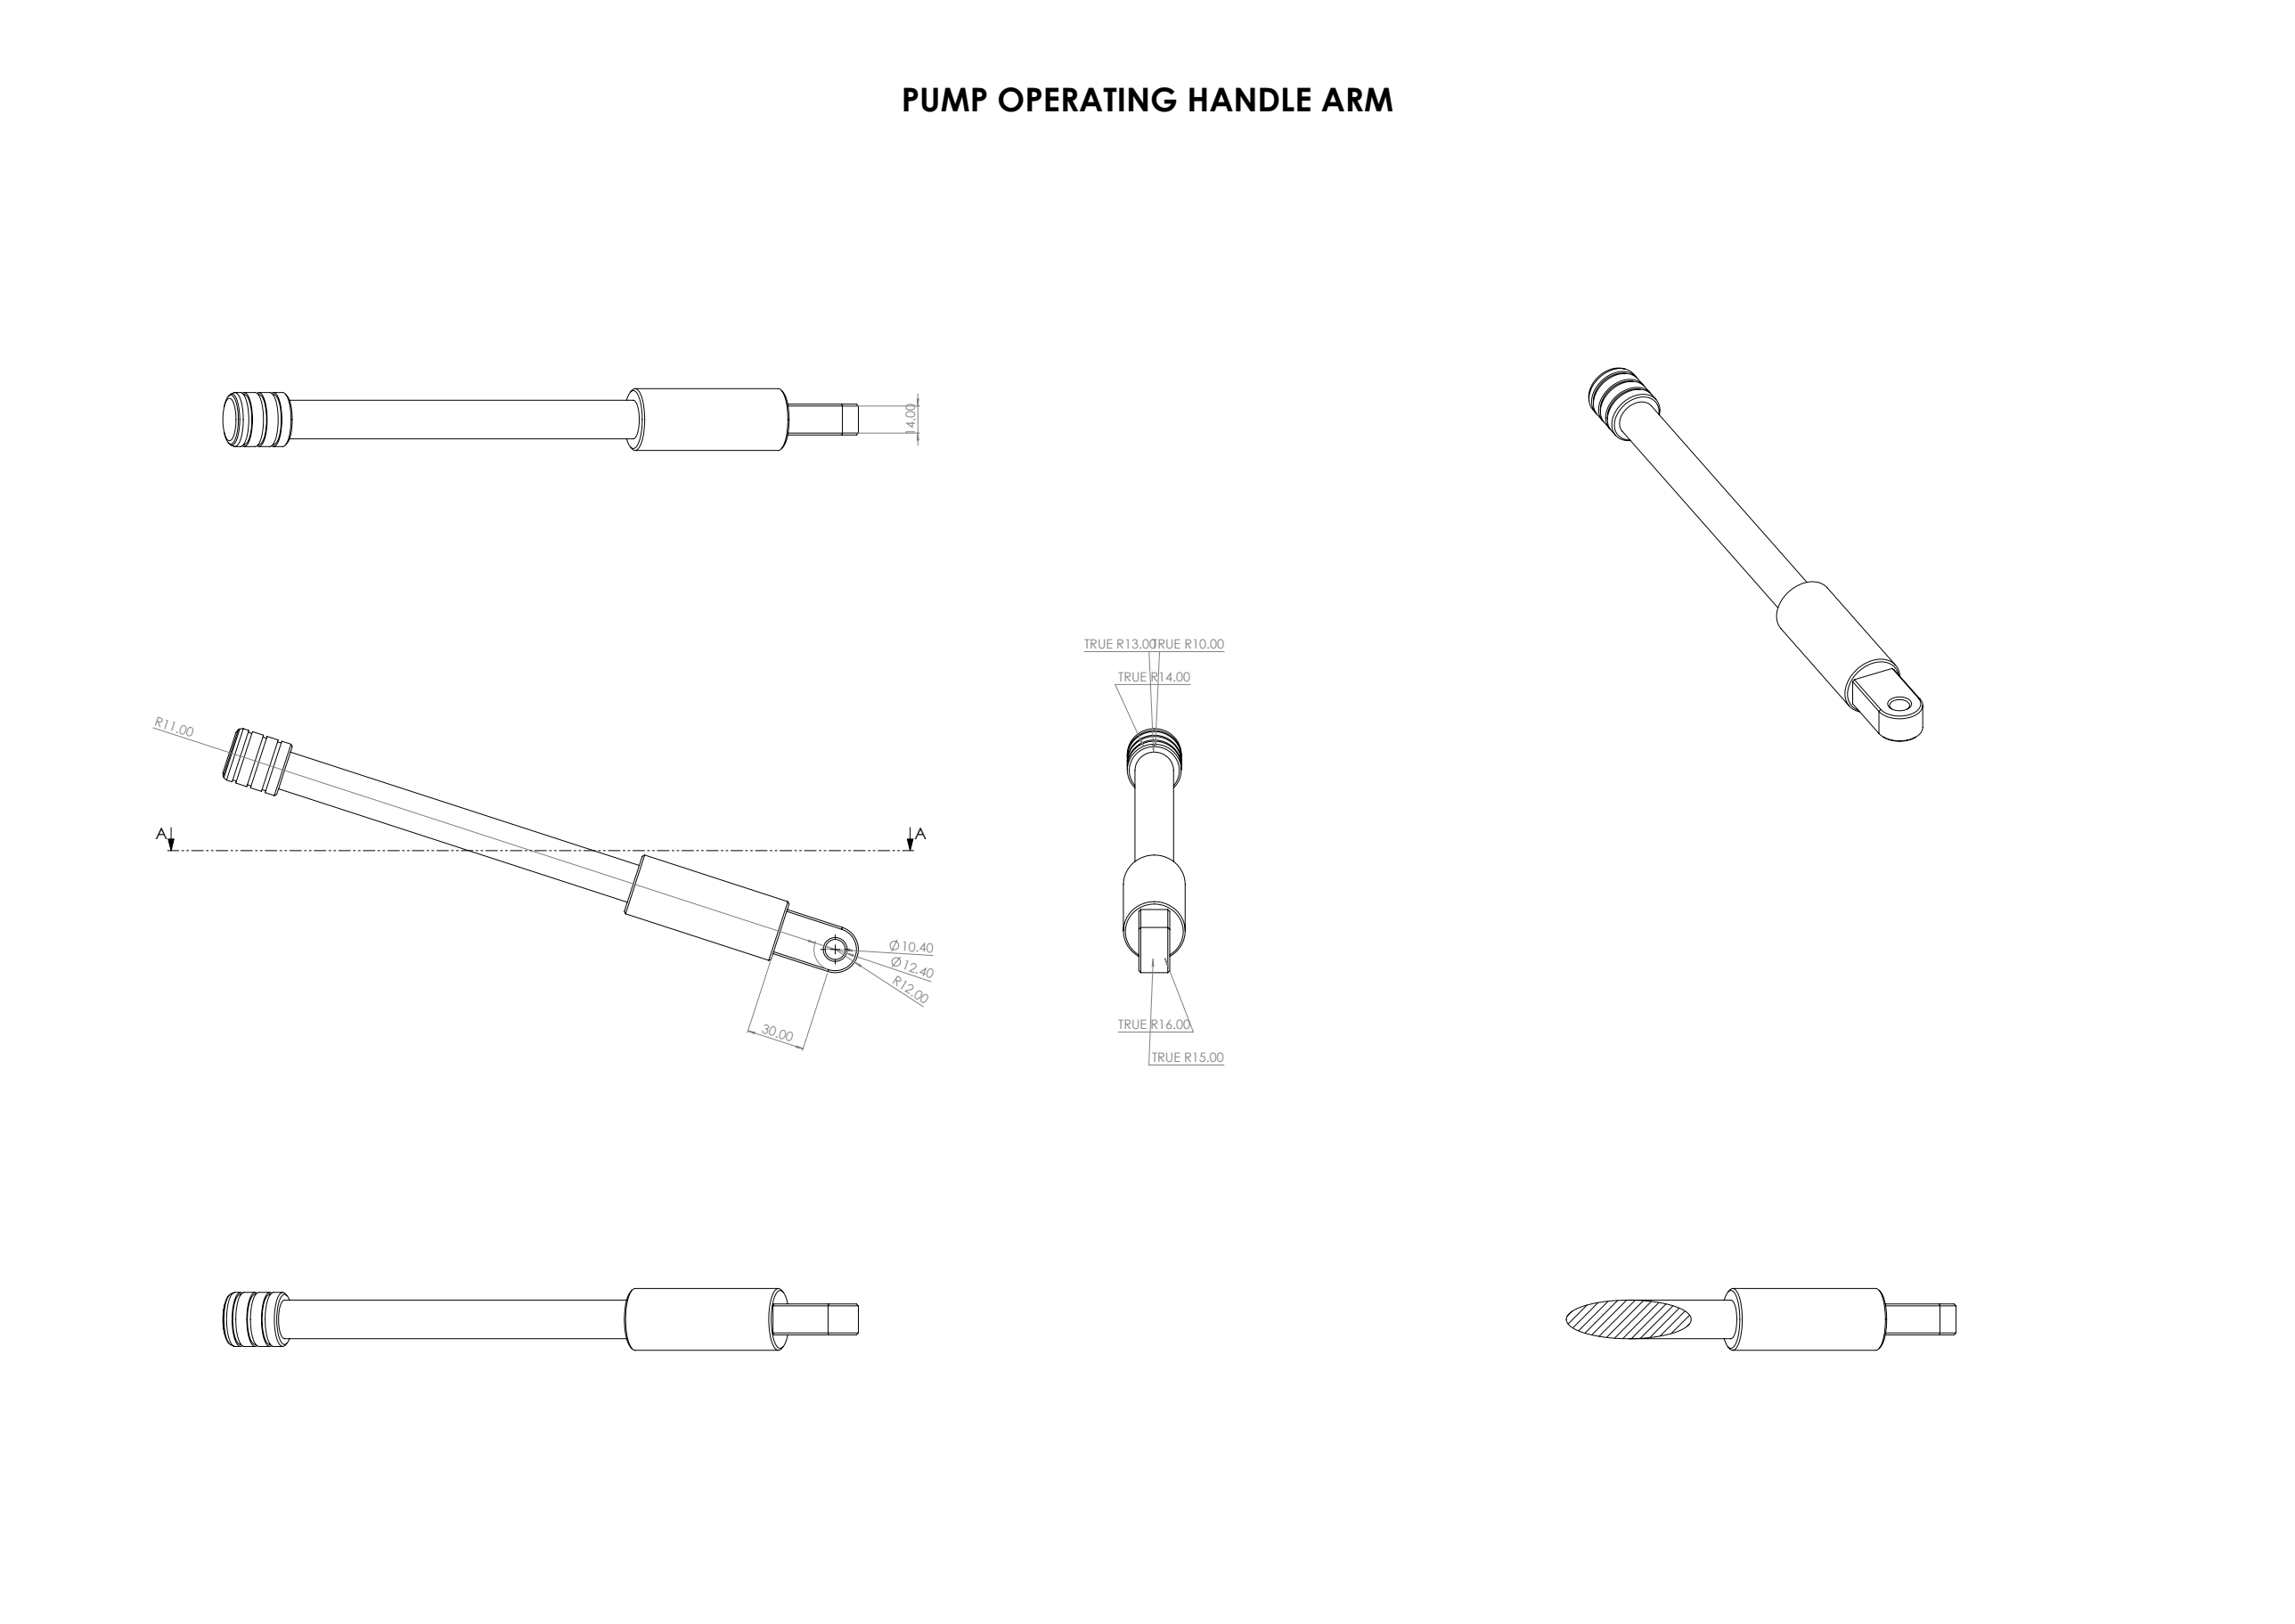
ISO-10303-21;
HEADER;
/* Generated by software containing ST-Developer
 * from STEP Tools, Inc. (www.steptools.com) 
 */

FILE_DESCRIPTION(
/* description */ (''),
/* implementation_level */ '2;1');

FILE_NAME(
/* name */ '11_Pump_Operating_Handle_Arm.step',
/* time_stamp */ '2026-10-20T10:03:03-07:00',
/* author */ (''),
/* organization */ (''),
/* preprocessor_version */ 'ST-DEVELOPER v20.2',
/* originating_system */ 'Autodesk Translation Framework v15.15.0.0',
/* authorisation */ '');

FILE_SCHEMA (('AUTOMOTIVE_DESIGN { 1 0 10303 214 3 1 1 }'));
ENDSEC;

DATA;
#10=MECHANICAL_DESIGN_GEOMETRIC_PRESENTATION_REPRESENTATION('',(#542,#543,#544,#545,#546,#547,#548,#549),#71492);
#399=SHAPE_REPRESENTATION_RELATIONSHIP('SRR','None',#71620,#418);
#418=ADVANCED_BREP_SHAPE_REPRESENTATION('',(#437),#71490);
#437=MANIFOLD_SOLID_BREP('Handle',#28476);
#542=STYLED_ITEM('',(#71880),#28308);
#543=STYLED_ITEM('',(#71880),#28315);
#544=STYLED_ITEM('',(#71880),#28318);
#545=STYLED_ITEM('',(#71880),#28320);
#546=STYLED_ITEM('',(#71880),#28322);
#547=STYLED_ITEM('',(#71880),#28324);
#548=STYLED_ITEM('',(#71880),#28326);
#549=STYLED_ITEM('',(#71880),#437);
#1833=CYLINDRICAL_SURFACE('',#30489,1.40000000000001);
#1834=CYLINDRICAL_SURFACE('',#30494,0.52);
#1835=CYLINDRICAL_SURFACE('',#30506,1.40000000000001);
#1836=CYLINDRICAL_SURFACE('',#30512,1.30000000000003);
#1837=CYLINDRICAL_SURFACE('',#30516,1.40000000000001);
#1838=CYLINDRICAL_SURFACE('',#30520,1.3);
#1839=CYLINDRICAL_SURFACE('',#30524,1.40000000000001);
#1840=CYLINDRICAL_SURFACE('',#30528,1.30000000000003);
#1841=CYLINDRICAL_SURFACE('',#30535,1.60000000000001);
#1842=CYLINDRICAL_SURFACE('',#30541,0.999999999999985);
#1843=CYLINDRICAL_SURFACE('',#30548,1.19999999999999);
#1988=FACE_BOUND('',#6098,.T.);
#1989=FACE_BOUND('',#6101,.T.);
#1990=FACE_BOUND('',#6105,.T.);
#1991=FACE_BOUND('',#6107,.T.);
#1992=FACE_BOUND('',#6110,.T.);
#1993=FACE_BOUND('',#6113,.T.);
#1994=FACE_BOUND('',#6116,.T.);
#1995=FACE_BOUND('',#6119,.T.);
#1996=FACE_BOUND('',#6122,.T.);
#1997=FACE_BOUND('',#6124,.T.);
#1998=FACE_BOUND('',#6129,.T.);
#2575=CIRCLE('',#30479,1.1);
#2576=CIRCLE('',#30480,1.27071067811866);
#2577=CIRCLE('',#30481,1.27071067811866);
#2578=CIRCLE('',#30483,1.32928932188137);
#2579=CIRCLE('',#30484,1.32928932188137);
#2580=CIRCLE('',#30487,1.40000000000001);
#2581=CIRCLE('',#30488,1.40000000000001);
#2582=CIRCLE('',#30490,1.40000000000001);
#2583=CIRCLE('',#30492,0.619999999999999);
#2584=CIRCLE('',#30493,0.52);
#2585=CIRCLE('',#30495,0.52);
#2586=CIRCLE('',#30497,1.09999999999999);
#2587=CIRCLE('',#30499,0.619999999999999);
#2588=CIRCLE('',#30501,1.09999999999999);
#2589=CIRCLE('',#30503,1.40000000000001);
#2590=CIRCLE('',#30504,1.40000000000001);
#2591=CIRCLE('',#30505,1.30000000000001);
#2592=CIRCLE('',#30507,1.40000000000001);
#2593=CIRCLE('',#30509,1.);
#2594=CIRCLE('',#30511,1.30000000000002);
#2595=CIRCLE('',#30513,1.30000000000002);
#2596=CIRCLE('',#30515,1.40000000000001);
#2597=CIRCLE('',#30517,1.40000000000001);
#2598=CIRCLE('',#30519,1.29999999999999);
#2599=CIRCLE('',#30521,1.29999999999999);
#2600=CIRCLE('',#30523,1.40000000000001);
#2601=CIRCLE('',#30525,1.40000000000001);
#2602=CIRCLE('',#30527,1.30000000000002);
#2603=CIRCLE('',#30529,1.30000000000002);
#2604=CIRCLE('',#30532,1.5);
#2605=CIRCLE('',#30534,1.6);
#2606=CIRCLE('',#30536,1.60000000000002);
#2607=CIRCLE('',#30538,1.5);
#2608=CIRCLE('',#30540,0.999999999999996);
#2609=CIRCLE('',#30546,1.19999999999999);
#2610=CIRCLE('',#30549,1.19999999999999);
#2901=CONICAL_SURFACE('',#30478,1.18535533905933,1.17809724509622);
#2902=CONICAL_SURFACE('',#30482,1.30000000000001,0.78539816339746);
#2903=CONICAL_SURFACE('',#30486,1.36464466094069,0.392699081698615);
#2904=CONICAL_SURFACE('',#30491,0.569999999999999,0.785398163397448);
#2905=CONICAL_SURFACE('',#30498,0.569999999999999,0.785398163397448);
#2906=CONICAL_SURFACE('',#30502,1.35000000000001,0.785398163397418);
#2907=CONICAL_SURFACE('',#30533,1.54999999999999,0.785398163397423);
#2908=CONICAL_SURFACE('',#30537,1.54999999999999,0.785398163397517);
#2909=CONICAL_SURFACE('',#30545,1.14999999999999,0.785398163397454);
#2910=CONICAL_SURFACE('',#30551,1.14999999999999,0.785398163397454);
#4396=FACE_OUTER_BOUND('',#6090,.T.);
#4397=FACE_OUTER_BOUND('',#6091,.T.);
#4398=FACE_OUTER_BOUND('',#6092,.T.);
#4399=FACE_OUTER_BOUND('',#6093,.T.);
#4400=FACE_OUTER_BOUND('',#6094,.T.);
#4401=FACE_OUTER_BOUND('',#6095,.T.);
#4402=FACE_OUTER_BOUND('',#6096,.T.);
#4403=FACE_OUTER_BOUND('',#6097,.T.);
#4404=FACE_OUTER_BOUND('',#6099,.T.);
#4405=FACE_OUTER_BOUND('',#6100,.T.);
#4406=FACE_OUTER_BOUND('',#6102,.T.);
#4407=FACE_OUTER_BOUND('',#6103,.T.);
#4408=FACE_OUTER_BOUND('',#6104,.T.);
#4409=FACE_OUTER_BOUND('',#6106,.T.);
#4410=FACE_OUTER_BOUND('',#6108,.T.);
#4411=FACE_OUTER_BOUND('',#6109,.T.);
#4412=FACE_OUTER_BOUND('',#6111,.T.);
#4413=FACE_OUTER_BOUND('',#6112,.T.);
#4414=FACE_OUTER_BOUND('',#6114,.T.);
#4415=FACE_OUTER_BOUND('',#6115,.T.);
#4416=FACE_OUTER_BOUND('',#6117,.T.);
#4417=FACE_OUTER_BOUND('',#6118,.T.);
#4418=FACE_OUTER_BOUND('',#6120,.T.);
#4419=FACE_OUTER_BOUND('',#6121,.T.);
#4420=FACE_OUTER_BOUND('',#6123,.T.);
#4421=FACE_OUTER_BOUND('',#6125,.T.);
#4422=FACE_OUTER_BOUND('',#6126,.T.);
#4423=FACE_OUTER_BOUND('',#6127,.T.);
#4424=FACE_OUTER_BOUND('',#6128,.T.);
#4425=FACE_OUTER_BOUND('',#6130,.T.);
#4426=FACE_OUTER_BOUND('',#6131,.T.);
#4427=FACE_OUTER_BOUND('',#6132,.T.);
#4428=FACE_OUTER_BOUND('',#6133,.T.);
#4429=FACE_OUTER_BOUND('',#6134,.T.);
#4430=FACE_OUTER_BOUND('',#6135,.T.);
#4431=FACE_OUTER_BOUND('',#6136,.T.);
#4432=FACE_OUTER_BOUND('',#6137,.T.);
#4433=FACE_OUTER_BOUND('',#6138,.T.);
#4434=FACE_OUTER_BOUND('',#6139,.T.);
#6090=EDGE_LOOP('',(#25387,#25388,#25389,#25390,#25391));
#6091=EDGE_LOOP('',(#25392,#25393,#25394,#25395,#25396,#25397));
#6092=EDGE_LOOP('',(#25398));
#6093=EDGE_LOOP('',(#25399,#25400,#25401,#25402,#25403,#25404));
#6094=EDGE_LOOP('',(#25405,#25406,#25407,#25408,#25409));
#6095=EDGE_LOOP('',(#25410,#25411,#25412,#25413));
#6096=EDGE_LOOP('',(#25414,#25415,#25416,#25417));
#6097=EDGE_LOOP('',(#25418,#25419,#25420,#25421));
#6098=EDGE_LOOP('',(#25422));
#6099=EDGE_LOOP('',(#25423,#25424,#25425,#25426));
#6100=EDGE_LOOP('',(#25427,#25428,#25429,#25430));
#6101=EDGE_LOOP('',(#25431));
#6102=EDGE_LOOP('',(#25432,#25433,#25434,#25435,#25436));
#6103=EDGE_LOOP('',(#25437,#25438,#25439,#25440,#25441));
#6104=EDGE_LOOP('',(#25442));
#6105=EDGE_LOOP('',(#25443));
#6106=EDGE_LOOP('',(#25444));
#6107=EDGE_LOOP('',(#25445));
#6108=EDGE_LOOP('',(#25446,#25447,#25448,#25449));
#6109=EDGE_LOOP('',(#25450));
#6110=EDGE_LOOP('',(#25451));
#6111=EDGE_LOOP('',(#25452,#25453,#25454,#25455));
#6112=EDGE_LOOP('',(#25456));
#6113=EDGE_LOOP('',(#25457));
#6114=EDGE_LOOP('',(#25458,#25459,#25460,#25461));
#6115=EDGE_LOOP('',(#25462));
#6116=EDGE_LOOP('',(#25463));
#6117=EDGE_LOOP('',(#25464,#25465,#25466,#25467));
#6118=EDGE_LOOP('',(#25468));
#6119=EDGE_LOOP('',(#25469));
#6120=EDGE_LOOP('',(#25470,#25471,#25472,#25473));
#6121=EDGE_LOOP('',(#25474));
#6122=EDGE_LOOP('',(#25475));
#6123=EDGE_LOOP('',(#25476));
#6124=EDGE_LOOP('',(#25477,#25478,#25479,#25480,#25481,#25482,#25483,#25484));
#6125=EDGE_LOOP('',(#25485,#25486,#25487,#25488));
#6126=EDGE_LOOP('',(#25489,#25490,#25491,#25492));
#6127=EDGE_LOOP('',(#25493,#25494,#25495,#25496));
#6128=EDGE_LOOP('',(#25497));
#6129=EDGE_LOOP('',(#25498));
#6130=EDGE_LOOP('',(#25499,#25500,#25501,#25502));
#6131=EDGE_LOOP('',(#25503,#25504,#25505,#25506));
#6132=EDGE_LOOP('',(#25507,#25508,#25509,#25510));
#6133=EDGE_LOOP('',(#25511,#25512,#25513,#25514));
#6134=EDGE_LOOP('',(#25515,#25516,#25517,#25518));
#6135=EDGE_LOOP('',(#25519,#25520,#25521,#25522));
#6136=EDGE_LOOP('',(#25523,#25524,#25525,#25526));
#6137=EDGE_LOOP('',(#25527,#25528,#25529,#25530));
#6138=EDGE_LOOP('',(#25531,#25532,#25533,#25534));
#6139=EDGE_LOOP('',(#25535,#25536,#25537,#25538));
#8604=LINE('',#70692,#11092);
#8605=LINE('',#70698,#11093);
#8606=LINE('',#70705,#11094);
#8607=LINE('',#70711,#11095);
#8608=LINE('',#70717,#11096);
#8609=LINE('',#70722,#11097);
#8610=LINE('',#70726,#11098);
#8611=LINE('',#70728,#11099);
#8612=LINE('',#70731,#11100);
#8613=LINE('',#70735,#11101);
#8614=LINE('',#70739,#11102);
#8615=LINE('',#70741,#11103);
#8616=LINE('',#70744,#11104);
#8617=LINE('',#70751,#11105);
#8618=LINE('',#70756,#11106);
#8619=LINE('',#70766,#11107);
#8620=LINE('',#70772,#11108);
#8621=LINE('',#70780,#11109);
#8622=LINE('',#70786,#11110);
#8623=LINE('',#70794,#11111);
#8624=LINE('',#70800,#11112);
#8625=LINE('',#70802,#11113);
#8626=LINE('',#70804,#11114);
#8627=LINE('',#70805,#11115);
#8628=LINE('',#70807,#11116);
#8629=LINE('',#70808,#11117);
#8630=LINE('',#70812,#11118);
#8631=LINE('',#70816,#11119);
#8632=LINE('',#70820,#11120);
#8633=LINE('',#70825,#11121);
#8634=LINE('',#70828,#11122);
#8635=LINE('',#70829,#11123);
#8636=LINE('',#70832,#11124);
#8637=LINE('',#70833,#11125);
#8638=LINE('',#70835,#11126);
#8639=LINE('',#70838,#11127);
#8640=LINE('',#70841,#11128);
#8641=LINE('',#70845,#11129);
#8642=LINE('',#70847,#11130);
#8643=LINE('',#70848,#11131);
#11092=VECTOR('',#36741,1.18535533905933);
#11093=VECTOR('',#36748,1.30000000000001);
#11094=VECTOR('',#36757,1.36464466094067);
#11095=VECTOR('',#36764,1.40000000000001);
#11096=VECTOR('',#36771,0.57);
#11097=VECTOR('',#36778,0.52);
#11098=VECTOR('',#36781,1.);
#11099=VECTOR('',#36782,1.);
#11100=VECTOR('',#36785,1.);
#11101=VECTOR('',#36790,0.57);
#11102=VECTOR('',#36793,1.);
#11103=VECTOR('',#36794,1.);
#11104=VECTOR('',#36797,1.);
#11105=VECTOR('',#36804,1.35000000000004);
#11106=VECTOR('',#36811,1.40000000000001);
#11107=VECTOR('',#36824,1.30000000000003);
#11108=VECTOR('',#36831,1.40000000000001);
#11109=VECTOR('',#36842,1.3);
#11110=VECTOR('',#36849,1.40000000000001);
#11111=VECTOR('',#36860,1.30000000000003);
#11112=VECTOR('',#36867,1.);
#11113=VECTOR('',#36868,1.);
#11114=VECTOR('',#36869,1.);
#11115=VECTOR('',#36870,1.);
#11116=VECTOR('',#36871,1.);
#11117=VECTOR('',#36872,1.);
#11118=VECTOR('',#36877,1.54999999999999);
#11119=VECTOR('',#36882,1.60000000000001);
#11120=VECTOR('',#36887,1.54999999999999);
#11121=VECTOR('',#36894,0.999999999999985);
#11122=VECTOR('',#36897,1.);
#11123=VECTOR('',#36898,1.);
#11124=VECTOR('',#36901,1.);
#11125=VECTOR('',#36902,1.);
#11126=VECTOR('',#36905,1.);
#11127=VECTOR('',#36908,1.);
#11128=VECTOR('',#36913,1.);
#11129=VECTOR('',#36918,1.);
#11130=VECTOR('',#36921,1.);
#11131=VECTOR('',#36922,1.);
#13643=VERTEX_POINT('',#70689);
#13644=VERTEX_POINT('',#70691);
#13645=VERTEX_POINT('',#70693);
#13646=VERTEX_POINT('',#70697);
#13647=VERTEX_POINT('',#70699);
#13648=VERTEX_POINT('',#70704);
#13649=VERTEX_POINT('',#70706);
#13650=VERTEX_POINT('',#70710);
#13651=VERTEX_POINT('',#70714);
#13652=VERTEX_POINT('',#70716);
#13653=VERTEX_POINT('',#70720);
#13654=VERTEX_POINT('',#70724);
#13655=VERTEX_POINT('',#70725);
#13656=VERTEX_POINT('',#70727);
#13657=VERTEX_POINT('',#70729);
#13658=VERTEX_POINT('',#70733);
#13659=VERTEX_POINT('',#70737);
#13660=VERTEX_POINT('',#70738);
#13661=VERTEX_POINT('',#70740);
#13662=VERTEX_POINT('',#70742);
#13663=VERTEX_POINT('',#70746);
#13664=VERTEX_POINT('',#70747);
#13665=VERTEX_POINT('',#70750);
#13666=VERTEX_POINT('',#70754);
#13667=VERTEX_POINT('',#70758);
#13668=VERTEX_POINT('',#70761);
#13669=VERTEX_POINT('',#70764);
#13670=VERTEX_POINT('',#70768);
#13671=VERTEX_POINT('',#70771);
#13672=VERTEX_POINT('',#70775);
#13673=VERTEX_POINT('',#70778);
#13674=VERTEX_POINT('',#70782);
#13675=VERTEX_POINT('',#70785);
#13676=VERTEX_POINT('',#70789);
#13677=VERTEX_POINT('',#70792);
#13678=VERTEX_POINT('',#70797);
#13679=VERTEX_POINT('',#70799);
#13680=VERTEX_POINT('',#70801);
#13681=VERTEX_POINT('',#70803);
#13682=VERTEX_POINT('',#70806);
#13683=VERTEX_POINT('',#70810);
#13684=VERTEX_POINT('',#70814);
#13685=VERTEX_POINT('',#70818);
#13686=VERTEX_POINT('',#70822);
#13687=VERTEX_POINT('',#70827);
#13688=VERTEX_POINT('',#70831);
#13689=VERTEX_POINT('',#70837);
#13690=VERTEX_POINT('',#70843);
#17577=EDGE_CURVE('',#13643,#13643,#2575,.T.);
#17578=EDGE_CURVE('',#13643,#13644,#8604,.T.);
#17579=EDGE_CURVE('',#13644,#13645,#2576,.T.);
#17580=EDGE_CURVE('',#13645,#13644,#2577,.T.);
#17581=EDGE_CURVE('',#13645,#13646,#8605,.T.);
#17582=EDGE_CURVE('',#13647,#13646,#2578,.T.);
#17583=EDGE_CURVE('',#13646,#13647,#2579,.T.);
#17584=EDGE_CURVE('',#13647,#13648,#8606,.T.);
#17585=EDGE_CURVE('',#13648,#13649,#2580,.T.);
#17586=EDGE_CURVE('',#13649,#13648,#2581,.T.);
#17587=EDGE_CURVE('',#13649,#13650,#8607,.T.);
#17588=EDGE_CURVE('',#13650,#13650,#2582,.T.);
#17589=EDGE_CURVE('',#13651,#13651,#2583,.T.);
#17590=EDGE_CURVE('',#13651,#13652,#8608,.T.);
#17591=EDGE_CURVE('',#13652,#13652,#2584,.T.);
#17592=EDGE_CURVE('',#13653,#13653,#2585,.T.);
#17593=EDGE_CURVE('',#13653,#13652,#8609,.T.);
#17594=EDGE_CURVE('',#13654,#13655,#8610,.T.);
#17595=EDGE_CURVE('',#13656,#13655,#8611,.T.);
#17596=EDGE_CURVE('',#13657,#13656,#2586,.T.);
#17597=EDGE_CURVE('',#13654,#13657,#8612,.T.);
#17598=EDGE_CURVE('',#13658,#13658,#2587,.T.);
#17599=EDGE_CURVE('',#13658,#13653,#8613,.T.);
#17600=EDGE_CURVE('',#13659,#13660,#8614,.T.);
#17601=EDGE_CURVE('',#13661,#13660,#8615,.T.);
#17602=EDGE_CURVE('',#13662,#13661,#2588,.T.);
#17603=EDGE_CURVE('',#13659,#13662,#8616,.T.);
#17604=EDGE_CURVE('',#13663,#13664,#2589,.T.);
#17605=EDGE_CURVE('',#13664,#13663,#2590,.T.);
#17606=EDGE_CURVE('',#13663,#13665,#8617,.T.);
#17607=EDGE_CURVE('',#13665,#13665,#2591,.T.);
#17608=EDGE_CURVE('',#13666,#13666,#2592,.T.);
#17609=EDGE_CURVE('',#13666,#13664,#8618,.T.);
#17610=EDGE_CURVE('',#13667,#13667,#2593,.T.);
#17611=EDGE_CURVE('',#13668,#13668,#2594,.T.);
#17612=EDGE_CURVE('',#13669,#13669,#2595,.T.);
#17613=EDGE_CURVE('',#13669,#13668,#8619,.T.);
#17614=EDGE_CURVE('',#13670,#13670,#2596,.T.);
#17615=EDGE_CURVE('',#13670,#13671,#8620,.T.);
#17616=EDGE_CURVE('',#13671,#13671,#2597,.T.);
#17617=EDGE_CURVE('',#13672,#13672,#2598,.T.);
#17618=EDGE_CURVE('',#13673,#13673,#2599,.T.);
#17619=EDGE_CURVE('',#13673,#13672,#8621,.T.);
#17620=EDGE_CURVE('',#13674,#13674,#2600,.T.);
#17621=EDGE_CURVE('',#13674,#13675,#8622,.T.);
#17622=EDGE_CURVE('',#13675,#13675,#2601,.T.);
#17623=EDGE_CURVE('',#13676,#13676,#2602,.T.);
#17624=EDGE_CURVE('',#13677,#13677,#2603,.T.);
#17625=EDGE_CURVE('',#13677,#13676,#8623,.T.);
#17626=EDGE_CURVE('',#13678,#13678,#2604,.T.);
#17627=EDGE_CURVE('',#13660,#13679,#8624,.T.);
#17628=EDGE_CURVE('',#13680,#13659,#8625,.T.);
#17629=EDGE_CURVE('',#13681,#13680,#8626,.T.);
#17630=EDGE_CURVE('',#13655,#13681,#8627,.T.);
#17631=EDGE_CURVE('',#13682,#13654,#8628,.T.);
#17632=EDGE_CURVE('',#13679,#13682,#8629,.T.);
#17633=EDGE_CURVE('',#13683,#13683,#2605,.T.);
#17634=EDGE_CURVE('',#13683,#13678,#8630,.T.);
#17635=EDGE_CURVE('',#13684,#13684,#2606,.T.);
#17636=EDGE_CURVE('',#13684,#13683,#8631,.T.);
#17637=EDGE_CURVE('',#13685,#13685,#2607,.T.);
#17638=EDGE_CURVE('',#13685,#13684,#8632,.T.);
#17639=EDGE_CURVE('',#13686,#13686,#2608,.T.);
#17640=EDGE_CURVE('',#13667,#13686,#8633,.T.);
#17641=EDGE_CURVE('',#13681,#13687,#8634,.T.);
#17642=EDGE_CURVE('',#13687,#13656,#8635,.T.);
#17643=EDGE_CURVE('',#13688,#13680,#8636,.T.);
#17644=EDGE_CURVE('',#13688,#13687,#8637,.T.);
#17645=EDGE_CURVE('',#13688,#13662,#8638,.T.);
#17646=EDGE_CURVE('',#13689,#13657,#8639,.T.);
#17647=EDGE_CURVE('',#13687,#13689,#2609,.T.);
#17648=EDGE_CURVE('',#13689,#13682,#8640,.T.);
#17649=EDGE_CURVE('',#13690,#13688,#2610,.T.);
#17650=EDGE_CURVE('',#13690,#13689,#8641,.T.);
#17651=EDGE_CURVE('',#13679,#13690,#8642,.T.);
#17652=EDGE_CURVE('',#13690,#13661,#8643,.T.);
#25387=ORIENTED_EDGE('',*,*,#17577,.T.);
#25388=ORIENTED_EDGE('',*,*,#17578,.T.);
#25389=ORIENTED_EDGE('',*,*,#17579,.T.);
#25390=ORIENTED_EDGE('',*,*,#17580,.T.);
#25391=ORIENTED_EDGE('',*,*,#17578,.F.);
#25392=ORIENTED_EDGE('',*,*,#17579,.F.);
#25393=ORIENTED_EDGE('',*,*,#17580,.F.);
#25394=ORIENTED_EDGE('',*,*,#17581,.T.);
#25395=ORIENTED_EDGE('',*,*,#17582,.F.);
#25396=ORIENTED_EDGE('',*,*,#17583,.F.);
#25397=ORIENTED_EDGE('',*,*,#17581,.F.);
#25398=ORIENTED_EDGE('',*,*,#17577,.F.);
#25399=ORIENTED_EDGE('',*,*,#17582,.T.);
#25400=ORIENTED_EDGE('',*,*,#17583,.T.);
#25401=ORIENTED_EDGE('',*,*,#17584,.T.);
#25402=ORIENTED_EDGE('',*,*,#17585,.T.);
#25403=ORIENTED_EDGE('',*,*,#17586,.T.);
#25404=ORIENTED_EDGE('',*,*,#17584,.F.);
#25405=ORIENTED_EDGE('',*,*,#17585,.F.);
#25406=ORIENTED_EDGE('',*,*,#17586,.F.);
#25407=ORIENTED_EDGE('',*,*,#17587,.T.);
#25408=ORIENTED_EDGE('',*,*,#17588,.T.);
#25409=ORIENTED_EDGE('',*,*,#17587,.F.);
#25410=ORIENTED_EDGE('',*,*,#17589,.T.);
#25411=ORIENTED_EDGE('',*,*,#17590,.T.);
#25412=ORIENTED_EDGE('',*,*,#17591,.T.);
#25413=ORIENTED_EDGE('',*,*,#17590,.F.);
#25414=ORIENTED_EDGE('',*,*,#17592,.F.);
#25415=ORIENTED_EDGE('',*,*,#17593,.T.);
#25416=ORIENTED_EDGE('',*,*,#17591,.F.);
#25417=ORIENTED_EDGE('',*,*,#17593,.F.);
#25418=ORIENTED_EDGE('',*,*,#17594,.T.);
#25419=ORIENTED_EDGE('',*,*,#17595,.F.);
#25420=ORIENTED_EDGE('',*,*,#17596,.F.);
#25421=ORIENTED_EDGE('',*,*,#17597,.F.);
#25422=ORIENTED_EDGE('',*,*,#17589,.F.);
#25423=ORIENTED_EDGE('',*,*,#17598,.T.);
#25424=ORIENTED_EDGE('',*,*,#17599,.T.);
#25425=ORIENTED_EDGE('',*,*,#17592,.T.);
#25426=ORIENTED_EDGE('',*,*,#17599,.F.);
#25427=ORIENTED_EDGE('',*,*,#17600,.T.);
#25428=ORIENTED_EDGE('',*,*,#17601,.F.);
#25429=ORIENTED_EDGE('',*,*,#17602,.F.);
#25430=ORIENTED_EDGE('',*,*,#17603,.F.);
#25431=ORIENTED_EDGE('',*,*,#17598,.F.);
#25432=ORIENTED_EDGE('',*,*,#17604,.T.);
#25433=ORIENTED_EDGE('',*,*,#17605,.T.);
#25434=ORIENTED_EDGE('',*,*,#17606,.T.);
#25435=ORIENTED_EDGE('',*,*,#17607,.T.);
#25436=ORIENTED_EDGE('',*,*,#17606,.F.);
#25437=ORIENTED_EDGE('',*,*,#17608,.T.);
#25438=ORIENTED_EDGE('',*,*,#17609,.T.);
#25439=ORIENTED_EDGE('',*,*,#17604,.F.);
#25440=ORIENTED_EDGE('',*,*,#17605,.F.);
#25441=ORIENTED_EDGE('',*,*,#17609,.F.);
#25442=ORIENTED_EDGE('',*,*,#17607,.F.);
#25443=ORIENTED_EDGE('',*,*,#17610,.T.);
#25444=ORIENTED_EDGE('',*,*,#17588,.F.);
#25445=ORIENTED_EDGE('',*,*,#17611,.T.);
#25446=ORIENTED_EDGE('',*,*,#17612,.T.);
#25447=ORIENTED_EDGE('',*,*,#17613,.T.);
#25448=ORIENTED_EDGE('',*,*,#17611,.F.);
#25449=ORIENTED_EDGE('',*,*,#17613,.F.);
#25450=ORIENTED_EDGE('',*,*,#17614,.F.);
#25451=ORIENTED_EDGE('',*,*,#17612,.F.);
#25452=ORIENTED_EDGE('',*,*,#17614,.T.);
#25453=ORIENTED_EDGE('',*,*,#17615,.T.);
#25454=ORIENTED_EDGE('',*,*,#17616,.T.);
#25455=ORIENTED_EDGE('',*,*,#17615,.F.);
#25456=ORIENTED_EDGE('',*,*,#17616,.F.);
#25457=ORIENTED_EDGE('',*,*,#17617,.T.);
#25458=ORIENTED_EDGE('',*,*,#17618,.T.);
#25459=ORIENTED_EDGE('',*,*,#17619,.T.);
#25460=ORIENTED_EDGE('',*,*,#17617,.F.);
#25461=ORIENTED_EDGE('',*,*,#17619,.F.);
#25462=ORIENTED_EDGE('',*,*,#17620,.F.);
#25463=ORIENTED_EDGE('',*,*,#17618,.F.);
#25464=ORIENTED_EDGE('',*,*,#17620,.T.);
#25465=ORIENTED_EDGE('',*,*,#17621,.T.);
#25466=ORIENTED_EDGE('',*,*,#17622,.T.);
#25467=ORIENTED_EDGE('',*,*,#17621,.F.);
#25468=ORIENTED_EDGE('',*,*,#17622,.F.);
#25469=ORIENTED_EDGE('',*,*,#17623,.T.);
#25470=ORIENTED_EDGE('',*,*,#17624,.T.);
#25471=ORIENTED_EDGE('',*,*,#17625,.T.);
#25472=ORIENTED_EDGE('',*,*,#17623,.F.);
#25473=ORIENTED_EDGE('',*,*,#17625,.F.);
#25474=ORIENTED_EDGE('',*,*,#17608,.F.);
#25475=ORIENTED_EDGE('',*,*,#17624,.F.);
#25476=ORIENTED_EDGE('',*,*,#17626,.F.);
#25477=ORIENTED_EDGE('',*,*,#17627,.F.);
#25478=ORIENTED_EDGE('',*,*,#17600,.F.);
#25479=ORIENTED_EDGE('',*,*,#17628,.F.);
#25480=ORIENTED_EDGE('',*,*,#17629,.F.);
#25481=ORIENTED_EDGE('',*,*,#17630,.F.);
#25482=ORIENTED_EDGE('',*,*,#17594,.F.);
#25483=ORIENTED_EDGE('',*,*,#17631,.F.);
#25484=ORIENTED_EDGE('',*,*,#17632,.F.);
#25485=ORIENTED_EDGE('',*,*,#17633,.F.);
#25486=ORIENTED_EDGE('',*,*,#17634,.T.);
#25487=ORIENTED_EDGE('',*,*,#17626,.T.);
#25488=ORIENTED_EDGE('',*,*,#17634,.F.);
#25489=ORIENTED_EDGE('',*,*,#17635,.F.);
#25490=ORIENTED_EDGE('',*,*,#17636,.T.);
#25491=ORIENTED_EDGE('',*,*,#17633,.T.);
#25492=ORIENTED_EDGE('',*,*,#17636,.F.);
#25493=ORIENTED_EDGE('',*,*,#17637,.F.);
#25494=ORIENTED_EDGE('',*,*,#17638,.T.);
#25495=ORIENTED_EDGE('',*,*,#17635,.T.);
#25496=ORIENTED_EDGE('',*,*,#17638,.F.);
#25497=ORIENTED_EDGE('',*,*,#17637,.T.);
#25498=ORIENTED_EDGE('',*,*,#17639,.F.);
#25499=ORIENTED_EDGE('',*,*,#17610,.F.);
#25500=ORIENTED_EDGE('',*,*,#17640,.T.);
#25501=ORIENTED_EDGE('',*,*,#17639,.T.);
#25502=ORIENTED_EDGE('',*,*,#17640,.F.);
#25503=ORIENTED_EDGE('',*,*,#17630,.T.);
#25504=ORIENTED_EDGE('',*,*,#17641,.T.);
#25505=ORIENTED_EDGE('',*,*,#17642,.T.);
#25506=ORIENTED_EDGE('',*,*,#17595,.T.);
#25507=ORIENTED_EDGE('',*,*,#17629,.T.);
#25508=ORIENTED_EDGE('',*,*,#17643,.F.);
#25509=ORIENTED_EDGE('',*,*,#17644,.T.);
#25510=ORIENTED_EDGE('',*,*,#17641,.F.);
#25511=ORIENTED_EDGE('',*,*,#17628,.T.);
#25512=ORIENTED_EDGE('',*,*,#17603,.T.);
#25513=ORIENTED_EDGE('',*,*,#17645,.F.);
#25514=ORIENTED_EDGE('',*,*,#17643,.T.);
#25515=ORIENTED_EDGE('',*,*,#17646,.T.);
#25516=ORIENTED_EDGE('',*,*,#17596,.T.);
#25517=ORIENTED_EDGE('',*,*,#17642,.F.);
#25518=ORIENTED_EDGE('',*,*,#17647,.T.);
#25519=ORIENTED_EDGE('',*,*,#17631,.T.);
#25520=ORIENTED_EDGE('',*,*,#17597,.T.);
#25521=ORIENTED_EDGE('',*,*,#17646,.F.);
#25522=ORIENTED_EDGE('',*,*,#17648,.T.);
#25523=ORIENTED_EDGE('',*,*,#17647,.F.);
#25524=ORIENTED_EDGE('',*,*,#17644,.F.);
#25525=ORIENTED_EDGE('',*,*,#17649,.F.);
#25526=ORIENTED_EDGE('',*,*,#17650,.T.);
#25527=ORIENTED_EDGE('',*,*,#17627,.T.);
#25528=ORIENTED_EDGE('',*,*,#17651,.T.);
#25529=ORIENTED_EDGE('',*,*,#17652,.T.);
#25530=ORIENTED_EDGE('',*,*,#17601,.T.);
#25531=ORIENTED_EDGE('',*,*,#17652,.F.);
#25532=ORIENTED_EDGE('',*,*,#17649,.T.);
#25533=ORIENTED_EDGE('',*,*,#17645,.T.);
#25534=ORIENTED_EDGE('',*,*,#17602,.T.);
#25535=ORIENTED_EDGE('',*,*,#17632,.T.);
#25536=ORIENTED_EDGE('',*,*,#17648,.F.);
#25537=ORIENTED_EDGE('',*,*,#17650,.F.);
#25538=ORIENTED_EDGE('',*,*,#17651,.F.);
#26835=PLANE('',#30485);
#26836=PLANE('',#30496);
#26837=PLANE('',#30500);
#26838=PLANE('',#30508);
#26839=PLANE('',#30510);
#26840=PLANE('',#30514);
#26841=PLANE('',#30518);
#26842=PLANE('',#30522);
#26843=PLANE('',#30526);
#26844=PLANE('',#30530);
#26845=PLANE('',#30531);
#26846=PLANE('',#30539);
#26847=PLANE('',#30542);
#26848=PLANE('',#30543);
#26849=PLANE('',#30544);
#26850=PLANE('',#30547);
#26851=PLANE('',#30550);
#26852=PLANE('',#30552);
#28304=ADVANCED_FACE('',(#4396),#2901,.T.);
#28305=ADVANCED_FACE('',(#4397),#2902,.T.);
#28306=ADVANCED_FACE('',(#4398),#26835,.T.);
#28307=ADVANCED_FACE('',(#4399),#2903,.T.);
#28308=ADVANCED_FACE('',(#4400),#1833,.T.);
#28309=ADVANCED_FACE('',(#4401),#2904,.F.);
#28310=ADVANCED_FACE('',(#4402),#1834,.F.);
#28311=ADVANCED_FACE('',(#4403,#1988),#26836,.T.);
#28312=ADVANCED_FACE('',(#4404),#2905,.F.);
#28313=ADVANCED_FACE('',(#4405,#1989),#26837,.F.);
#28314=ADVANCED_FACE('',(#4406),#2906,.T.);
#28315=ADVANCED_FACE('',(#4407),#1835,.T.);
#28316=ADVANCED_FACE('',(#4408,#1990),#26838,.T.);
#28317=ADVANCED_FACE('',(#4409,#1991),#26839,.F.);
#28318=ADVANCED_FACE('',(#4410),#1836,.T.);
#28319=ADVANCED_FACE('',(#4411,#1992),#26840,.F.);
#28320=ADVANCED_FACE('',(#4412),#1837,.T.);
#28321=ADVANCED_FACE('',(#4413,#1993),#26841,.F.);
#28322=ADVANCED_FACE('',(#4414),#1838,.T.);
#28323=ADVANCED_FACE('',(#4415,#1994),#26842,.F.);
#28324=ADVANCED_FACE('',(#4416),#1839,.T.);
#28325=ADVANCED_FACE('',(#4417,#1995),#26843,.F.);
#28326=ADVANCED_FACE('',(#4418),#1840,.T.);
#28327=ADVANCED_FACE('',(#4419,#1996),#26844,.F.);
#28328=ADVANCED_FACE('',(#4420,#1997),#26845,.T.);
#28329=ADVANCED_FACE('',(#4421),#2907,.T.);
#28330=ADVANCED_FACE('',(#4422),#1841,.T.);
#28331=ADVANCED_FACE('',(#4423),#2908,.T.);
#28332=ADVANCED_FACE('',(#4424,#1998),#26846,.T.);
#28333=ADVANCED_FACE('',(#4425),#1842,.T.);
#28334=ADVANCED_FACE('',(#4426),#26847,.T.);
#28335=ADVANCED_FACE('',(#4427),#26848,.T.);
#28336=ADVANCED_FACE('',(#4428),#26849,.T.);
#28337=ADVANCED_FACE('',(#4429),#2909,.T.);
#28338=ADVANCED_FACE('',(#4430),#26850,.T.);
#28339=ADVANCED_FACE('',(#4431),#1843,.T.);
#28340=ADVANCED_FACE('',(#4432),#26851,.T.);
#28341=ADVANCED_FACE('',(#4433),#2910,.T.);
#28342=ADVANCED_FACE('',(#4434),#26852,.T.);
#28476=CLOSED_SHELL('',(#28304,#28305,#28306,#28307,#28308,#28309,#28310,
#28311,#28312,#28313,#28314,#28315,#28316,#28317,#28318,#28319,#28320,#28321,
#28322,#28323,#28324,#28325,#28326,#28327,#28328,#28329,#28330,#28331,#28332,
#28333,#28334,#28335,#28336,#28337,#28338,#28339,#28340,#28341,#28342));
#30477=AXIS2_PLACEMENT_3D('',#70687,#36735,#36736);
#30478=AXIS2_PLACEMENT_3D('',#70688,#36737,#36738);
#30479=AXIS2_PLACEMENT_3D('',#70690,#36739,#36740);
#30480=AXIS2_PLACEMENT_3D('',#70694,#36742,#36743);
#30481=AXIS2_PLACEMENT_3D('',#70695,#36744,#36745);
#30482=AXIS2_PLACEMENT_3D('',#70696,#36746,#36747);
#30483=AXIS2_PLACEMENT_3D('',#70700,#36749,#36750);
#30484=AXIS2_PLACEMENT_3D('',#70701,#36751,#36752);
#30485=AXIS2_PLACEMENT_3D('',#70702,#36753,#36754);
#30486=AXIS2_PLACEMENT_3D('',#70703,#36755,#36756);
#30487=AXIS2_PLACEMENT_3D('',#70707,#36758,#36759);
#30488=AXIS2_PLACEMENT_3D('',#70708,#36760,#36761);
#30489=AXIS2_PLACEMENT_3D('',#70709,#36762,#36763);
#30490=AXIS2_PLACEMENT_3D('',#70712,#36765,#36766);
#30491=AXIS2_PLACEMENT_3D('',#70713,#36767,#36768);
#30492=AXIS2_PLACEMENT_3D('',#70715,#36769,#36770);
#30493=AXIS2_PLACEMENT_3D('',#70718,#36772,#36773);
#30494=AXIS2_PLACEMENT_3D('',#70719,#36774,#36775);
#30495=AXIS2_PLACEMENT_3D('',#70721,#36776,#36777);
#30496=AXIS2_PLACEMENT_3D('',#70723,#36779,#36780);
#30497=AXIS2_PLACEMENT_3D('',#70730,#36783,#36784);
#30498=AXIS2_PLACEMENT_3D('',#70732,#36786,#36787);
#30499=AXIS2_PLACEMENT_3D('',#70734,#36788,#36789);
#30500=AXIS2_PLACEMENT_3D('',#70736,#36791,#36792);
#30501=AXIS2_PLACEMENT_3D('',#70743,#36795,#36796);
#30502=AXIS2_PLACEMENT_3D('',#70745,#36798,#36799);
#30503=AXIS2_PLACEMENT_3D('',#70748,#36800,#36801);
#30504=AXIS2_PLACEMENT_3D('',#70749,#36802,#36803);
#30505=AXIS2_PLACEMENT_3D('',#70752,#36805,#36806);
#30506=AXIS2_PLACEMENT_3D('',#70753,#36807,#36808);
#30507=AXIS2_PLACEMENT_3D('',#70755,#36809,#36810);
#30508=AXIS2_PLACEMENT_3D('',#70757,#36812,#36813);
#30509=AXIS2_PLACEMENT_3D('',#70759,#36814,#36815);
#30510=AXIS2_PLACEMENT_3D('',#70760,#36816,#36817);
#30511=AXIS2_PLACEMENT_3D('',#70762,#36818,#36819);
#30512=AXIS2_PLACEMENT_3D('',#70763,#36820,#36821);
#30513=AXIS2_PLACEMENT_3D('',#70765,#36822,#36823);
#30514=AXIS2_PLACEMENT_3D('',#70767,#36825,#36826);
#30515=AXIS2_PLACEMENT_3D('',#70769,#36827,#36828);
#30516=AXIS2_PLACEMENT_3D('',#70770,#36829,#36830);
#30517=AXIS2_PLACEMENT_3D('',#70773,#36832,#36833);
#30518=AXIS2_PLACEMENT_3D('',#70774,#36834,#36835);
#30519=AXIS2_PLACEMENT_3D('',#70776,#36836,#36837);
#30520=AXIS2_PLACEMENT_3D('',#70777,#36838,#36839);
#30521=AXIS2_PLACEMENT_3D('',#70779,#36840,#36841);
#30522=AXIS2_PLACEMENT_3D('',#70781,#36843,#36844);
#30523=AXIS2_PLACEMENT_3D('',#70783,#36845,#36846);
#30524=AXIS2_PLACEMENT_3D('',#70784,#36847,#36848);
#30525=AXIS2_PLACEMENT_3D('',#70787,#36850,#36851);
#30526=AXIS2_PLACEMENT_3D('',#70788,#36852,#36853);
#30527=AXIS2_PLACEMENT_3D('',#70790,#36854,#36855);
#30528=AXIS2_PLACEMENT_3D('',#70791,#36856,#36857);
#30529=AXIS2_PLACEMENT_3D('',#70793,#36858,#36859);
#30530=AXIS2_PLACEMENT_3D('',#70795,#36861,#36862);
#30531=AXIS2_PLACEMENT_3D('',#70796,#36863,#36864);
#30532=AXIS2_PLACEMENT_3D('',#70798,#36865,#36866);
#30533=AXIS2_PLACEMENT_3D('',#70809,#36873,#36874);
#30534=AXIS2_PLACEMENT_3D('',#70811,#36875,#36876);
#30535=AXIS2_PLACEMENT_3D('',#70813,#36878,#36879);
#30536=AXIS2_PLACEMENT_3D('',#70815,#36880,#36881);
#30537=AXIS2_PLACEMENT_3D('',#70817,#36883,#36884);
#30538=AXIS2_PLACEMENT_3D('',#70819,#36885,#36886);
#30539=AXIS2_PLACEMENT_3D('',#70821,#36888,#36889);
#30540=AXIS2_PLACEMENT_3D('',#70823,#36890,#36891);
#30541=AXIS2_PLACEMENT_3D('',#70824,#36892,#36893);
#30542=AXIS2_PLACEMENT_3D('',#70826,#36895,#36896);
#30543=AXIS2_PLACEMENT_3D('',#70830,#36899,#36900);
#30544=AXIS2_PLACEMENT_3D('',#70834,#36903,#36904);
#30545=AXIS2_PLACEMENT_3D('',#70836,#36906,#36907);
#30546=AXIS2_PLACEMENT_3D('',#70839,#36909,#36910);
#30547=AXIS2_PLACEMENT_3D('',#70840,#36911,#36912);
#30548=AXIS2_PLACEMENT_3D('',#70842,#36914,#36915);
#30549=AXIS2_PLACEMENT_3D('',#70844,#36916,#36917);
#30550=AXIS2_PLACEMENT_3D('',#70846,#36919,#36920);
#30551=AXIS2_PLACEMENT_3D('',#70849,#36923,#36924);
#30552=AXIS2_PLACEMENT_3D('',#70850,#36925,#36926);
#36735=DIRECTION('axis',(0.,0.,1.));
#36736=DIRECTION('refdir',(1.,0.,0.));
#36737=DIRECTION('center_axis',(0.951056516295133,0.,0.309016994375011));
#36738=DIRECTION('ref_axis',(0.309016994374947,0.,-0.951056516295154));
#36739=DIRECTION('center_axis',(0.951056516295154,0.,0.309016994374948));
#36740=DIRECTION('ref_axis',(0.309016994374948,0.,-0.951056516295153));
#36741=DIRECTION('',(0.0784590957277245,1.13142611228773E-16,0.996917333733138));
#36742=DIRECTION('center_axis',(-0.951056516295154,-2.65900928743012E-15,
-0.309016994374947));
#36743=DIRECTION('ref_axis',(0.309016994374947,0.,-0.951056516295154));
#36744=DIRECTION('center_axis',(-0.951056516295154,-2.65900928743012E-15,
-0.309016994374947));
#36745=DIRECTION('ref_axis',(0.309016994374947,0.,-0.951056516295154));
#36746=DIRECTION('center_axis',(0.951056516295154,0.,0.309016994374948));
#36747=DIRECTION('ref_axis',(-0.309016994374944,0.,0.951056516295155));
#36748=DIRECTION('',(0.891006524188362,-8.65956056235505E-17,-0.453990499739558));
#36749=DIRECTION('center_axis',(0.951056516295154,0.,0.309016994374946));
#36750=DIRECTION('ref_axis',(0.309016994374946,0.,-0.951056516295154));
#36751=DIRECTION('center_axis',(0.951056516295154,0.,0.309016994374946));
#36752=DIRECTION('ref_axis',(0.309016994374946,0.,-0.951056516295154));
#36753=DIRECTION('center_axis',(-0.951056516295154,0.,-0.309016994374948));
#36754=DIRECTION('ref_axis',(-0.309016994374948,0.,0.951056516295154));
#36755=DIRECTION('center_axis',(0.951056516295153,0.,0.309016994374949));
#36756=DIRECTION('ref_axis',(0.309016994374945,0.,-0.951056516295154));
#36757=DIRECTION('',(0.760405965600097,4.68652040532512E-17,0.649448048330106));
#36758=DIRECTION('center_axis',(-0.951056516295154,0.,-0.309016994374948));
#36759=DIRECTION('ref_axis',(0.309016994374944,0.,-0.951056516295155));
#36760=DIRECTION('center_axis',(-0.951056516295154,0.,-0.309016994374948));
#36761=DIRECTION('ref_axis',(0.309016994374944,0.,-0.951056516295155));
#36762=DIRECTION('center_axis',(-0.951056516295154,0.,-0.309016994374948));
#36763=DIRECTION('ref_axis',(-0.309016994374944,0.,0.951056516295155));
#36764=DIRECTION('',(0.951056516295154,0.,0.309016994374948));
#36765=DIRECTION('center_axis',(-0.951056516295154,0.,-0.309016994374948));
#36766=DIRECTION('ref_axis',(-0.309016994374944,0.,0.951056516295155));
#36767=DIRECTION('center_axis',(0.,1.,0.));
#36768=DIRECTION('ref_axis',(1.,0.,0.));
#36769=DIRECTION('center_axis',(0.,1.,0.));
#36770=DIRECTION('ref_axis',(1.,0.,0.));
#36771=DIRECTION('',(0.707106781186547,-0.707106781186547,-8.65956056235493E-17));
#36772=DIRECTION('center_axis',(0.,-1.,0.));
#36773=DIRECTION('ref_axis',(1.,0.,0.));
#36774=DIRECTION('center_axis',(0.,1.,0.));
#36775=DIRECTION('ref_axis',(1.,0.,0.));
#36776=DIRECTION('center_axis',(0.,1.,0.));
#36777=DIRECTION('ref_axis',(1.,0.,0.));
#36778=DIRECTION('',(0.,1.,0.));
#36779=DIRECTION('center_axis',(0.,1.,0.));
#36780=DIRECTION('ref_axis',(1.,0.,0.));
#36781=DIRECTION('',(-0.309016994374948,0.,0.951056516295154));
#36782=DIRECTION('',(-0.951056516295154,0.,-0.309016994374947));
#36783=DIRECTION('center_axis',(0.,-1.,0.));
#36784=DIRECTION('ref_axis',(-0.309016994374959,0.,0.95105651629515));
#36785=DIRECTION('',(0.951056516295154,0.,0.309016994374947));
#36786=DIRECTION('center_axis',(0.,-1.,0.));
#36787=DIRECTION('ref_axis',(1.,0.,0.));
#36788=DIRECTION('center_axis',(0.,-1.,0.));
#36789=DIRECTION('ref_axis',(1.,0.,0.));
#36790=DIRECTION('',(0.707106781186547,0.707106781186547,8.65956056235493E-17));
#36791=DIRECTION('center_axis',(0.,1.,0.));
#36792=DIRECTION('ref_axis',(1.,0.,0.));
#36793=DIRECTION('',(0.309016994374948,0.,-0.951056516295154));
#36794=DIRECTION('',(-0.951056516295154,0.,-0.309016994374947));
#36795=DIRECTION('center_axis',(0.,1.,0.));
#36796=DIRECTION('ref_axis',(-0.309016994374959,0.,0.95105651629515));
#36797=DIRECTION('',(0.951056516295154,0.,0.309016994374947));
#36798=DIRECTION('center_axis',(-0.95105651629516,0.,-0.309016994374926));
#36799=DIRECTION('ref_axis',(0.309016994374946,0.,-0.951056516295154));
#36800=DIRECTION('center_axis',(0.951056516295154,0.,0.309016994374948));
#36801=DIRECTION('ref_axis',(0.309016994374944,0.,-0.951056516295155));
#36802=DIRECTION('center_axis',(0.951056516295154,0.,0.309016994374948));
#36803=DIRECTION('ref_axis',(0.309016994374944,0.,-0.951056516295155));
#36804=DIRECTION('',(0.891006524188383,-8.65956056235445E-17,-0.453990499739517));
#36805=DIRECTION('center_axis',(-0.951056516295154,0.,-0.309016994374948));
#36806=DIRECTION('ref_axis',(0.309016994374948,0.,-0.951056516295153));
#36807=DIRECTION('center_axis',(-0.951056516295154,0.,-0.309016994374948));
#36808=DIRECTION('ref_axis',(-0.309016994374944,0.,0.951056516295155));
#36809=DIRECTION('center_axis',(0.951056516295154,0.,0.309016994374948));
#36810=DIRECTION('ref_axis',(-0.309016994374944,0.,0.951056516295155));
#36811=DIRECTION('',(0.951056516295154,0.,0.309016994374948));
#36812=DIRECTION('center_axis',(0.951056516295154,0.,0.309016994374948));
#36813=DIRECTION('ref_axis',(0.309016994374948,0.,-0.951056516295154));
#36814=DIRECTION('center_axis',(-0.951056516295154,0.,-0.309016994374948));
#36815=DIRECTION('ref_axis',(0.309016994374948,0.,-0.951056516295154));
#36816=DIRECTION('center_axis',(-0.951056516295154,0.,-0.309016994374948));
#36817=DIRECTION('ref_axis',(-0.309016994374948,0.,0.951056516295154));
#36818=DIRECTION('center_axis',(-0.951056516295154,0.,-0.309016994374948));
#36819=DIRECTION('ref_axis',(0.309016994374948,0.,-0.951056516295154));
#36820=DIRECTION('center_axis',(-0.951056516295154,0.,-0.309016994374948));
#36821=DIRECTION('ref_axis',(-0.309016994374948,0.,0.951056516295153));
#36822=DIRECTION('center_axis',(-0.951056516295154,0.,-0.309016994374948));
#36823=DIRECTION('ref_axis',(0.309016994374948,0.,-0.951056516295154));
#36824=DIRECTION('',(-0.951056516295153,0.,-0.309016994374948));
#36825=DIRECTION('center_axis',(0.951056516295154,0.,0.309016994374948));
#36826=DIRECTION('ref_axis',(0.309016994374948,0.,-0.951056516295154));
#36827=DIRECTION('center_axis',(0.951056516295154,0.,0.309016994374948));
#36828=DIRECTION('ref_axis',(-0.309016994374944,0.,0.951056516295155));
#36829=DIRECTION('center_axis',(-0.951056516295154,0.,-0.309016994374948));
#36830=DIRECTION('ref_axis',(-0.309016994374944,0.,0.951056516295155));
#36831=DIRECTION('',(0.951056516295154,0.,0.309016994374948));
#36832=DIRECTION('center_axis',(-0.951056516295154,0.,-0.309016994374948));
#36833=DIRECTION('ref_axis',(-0.309016994374944,0.,0.951056516295155));
#36834=DIRECTION('center_axis',(-0.951056516295154,0.,-0.309016994374948));
#36835=DIRECTION('ref_axis',(-0.309016994374948,0.,0.951056516295154));
#36836=DIRECTION('center_axis',(-0.951056516295154,0.,-0.309016994374948));
#36837=DIRECTION('ref_axis',(0.309016994374948,0.,-0.951056516295153));
#36838=DIRECTION('center_axis',(-0.951056516295154,0.,-0.309016994374948));
#36839=DIRECTION('ref_axis',(-0.309016994374948,0.,0.951056516295154));
#36840=DIRECTION('center_axis',(-0.951056516295154,0.,-0.309016994374948));
#36841=DIRECTION('ref_axis',(0.309016994374948,0.,-0.951056516295153));
#36842=DIRECTION('',(-0.951056516295154,0.,-0.309016994374948));
#36843=DIRECTION('center_axis',(0.951056516295154,0.,0.309016994374948));
#36844=DIRECTION('ref_axis',(0.309016994374948,0.,-0.951056516295154));
#36845=DIRECTION('center_axis',(0.951056516295154,0.,0.309016994374948));
#36846=DIRECTION('ref_axis',(-0.309016994374944,0.,0.951056516295155));
#36847=DIRECTION('center_axis',(-0.951056516295154,0.,-0.309016994374948));
#36848=DIRECTION('ref_axis',(-0.309016994374944,0.,0.951056516295155));
#36849=DIRECTION('',(0.951056516295154,0.,0.309016994374948));
#36850=DIRECTION('center_axis',(-0.951056516295154,0.,-0.309016994374948));
#36851=DIRECTION('ref_axis',(-0.309016994374944,0.,0.951056516295155));
#36852=DIRECTION('center_axis',(-0.951056516295154,0.,-0.309016994374948));
#36853=DIRECTION('ref_axis',(-0.309016994374948,0.,0.951056516295154));
#36854=DIRECTION('center_axis',(-0.951056516295154,0.,-0.309016994374948));
#36855=DIRECTION('ref_axis',(0.309016994374948,0.,-0.951056516295154));
#36856=DIRECTION('center_axis',(-0.951056516295154,0.,-0.309016994374948));
#36857=DIRECTION('ref_axis',(-0.309016994374948,0.,0.951056516295153));
#36858=DIRECTION('center_axis',(-0.951056516295154,0.,-0.309016994374948));
#36859=DIRECTION('ref_axis',(0.309016994374948,0.,-0.951056516295154));
#36860=DIRECTION('',(-0.951056516295153,0.,-0.309016994374948));
#36861=DIRECTION('center_axis',(0.951056516295154,0.,0.309016994374948));
#36862=DIRECTION('ref_axis',(0.309016994374948,0.,-0.951056516295154));
#36863=DIRECTION('center_axis',(0.951056516295154,0.,0.309016994374948));
#36864=DIRECTION('ref_axis',(0.309016994374948,0.,-0.951056516295154));
#36865=DIRECTION('center_axis',(-0.951056516295154,0.,-0.309016994374948));
#36866=DIRECTION('ref_axis',(0.309016994374948,0.,-0.951056516295153));
#36867=DIRECTION('',(0.218508012224404,0.707106781186568,-0.672498511963937));
#36868=DIRECTION('',(0.218508012224404,-0.707106781186569,-0.672498511963937));
#36869=DIRECTION('',(0.,-1.,0.));
#36870=DIRECTION('',(-0.218508012224404,-0.707106781186569,0.672498511963937));
#36871=DIRECTION('',(-0.218508012224404,0.707106781186568,0.672498511963937));
#36872=DIRECTION('',(0.,1.,0.));
#36873=DIRECTION('center_axis',(-0.951056516295154,0.,-0.309016994374948));
#36874=DIRECTION('ref_axis',(-0.309016994374944,0.,0.951056516295155));
#36875=DIRECTION('center_axis',(-0.951056516295154,0.,-0.309016994374948));
#36876=DIRECTION('ref_axis',(0.309016994374948,0.,-0.951056516295153));
#36877=DIRECTION('',(0.453990499739571,8.6595605623547E-17,0.891006524188356));
#36878=DIRECTION('center_axis',(-0.951056516295154,0.,-0.309016994374948));
#36879=DIRECTION('ref_axis',(-0.309016994374944,0.,0.951056516295155));
#36880=DIRECTION('center_axis',(-0.951056516295154,0.,-0.309016994374948));
#36881=DIRECTION('ref_axis',(0.309016994374948,0.,-0.951056516295153));
#36882=DIRECTION('',(0.951056516295153,0.,0.309016994374948));
#36883=DIRECTION('center_axis',(0.951056516295154,0.,0.309016994374948));
#36884=DIRECTION('ref_axis',(-0.309016994374944,0.,0.951056516295155));
#36885=DIRECTION('center_axis',(-0.951056516295154,0.,-0.309016994374948));
#36886=DIRECTION('ref_axis',(0.309016994374948,0.,-0.951056516295154));
#36887=DIRECTION('',(0.891006524188336,-8.65956056235554E-17,-0.453990499739609));
#36888=DIRECTION('center_axis',(-0.951056516295154,0.,-0.309016994374948));
#36889=DIRECTION('ref_axis',(-0.309016994374948,0.,0.951056516295154));
#36890=DIRECTION('center_axis',(-0.951056516295154,0.,-0.309016994374948));
#36891=DIRECTION('ref_axis',(0.309016994374948,0.,-0.951056516295153));
#36892=DIRECTION('center_axis',(-0.951056516295154,0.,-0.309016994374948));
#36893=DIRECTION('ref_axis',(-0.309016994374944,0.,0.951056516295155));
#36894=DIRECTION('',(0.951056516295154,0.,0.309016994374948));
#36895=DIRECTION('center_axis',(-0.218508012224417,0.707106781186526,0.672498511963978));
#36896=DIRECTION('ref_axis',(0.951056516295154,0.,0.309016994374947));
#36897=DIRECTION('',(0.951056516295154,0.,0.309016994374947));
#36898=DIRECTION('',(0.218508012224407,0.707106781186617,-0.672498511963885));
#36899=DIRECTION('center_axis',(-0.309016994374947,0.,0.951056516295154));
#36900=DIRECTION('ref_axis',(0.951056516295154,0.,0.309016994374947));
#36901=DIRECTION('',(-0.951056516295154,0.,-0.309016994374947));
#36902=DIRECTION('',(0.,1.,0.));
#36903=DIRECTION('center_axis',(-0.218508012224417,-0.707106781186526,0.672498511963978));
#36904=DIRECTION('ref_axis',(0.951056516295154,0.,0.309016994374947));
#36905=DIRECTION('',(0.218508012224413,-0.707106781186516,-0.67249851196399));
#36906=DIRECTION('center_axis',(0.,-1.,0.));
#36907=DIRECTION('ref_axis',(-0.309016994374959,0.,0.95105651629515));
#36908=DIRECTION('',(-0.218508012224428,0.707106781186564,0.672498511963935));
#36909=DIRECTION('center_axis',(0.,1.,0.));
#36910=DIRECTION('ref_axis',(-0.309016994374959,0.,0.95105651629515));
#36911=DIRECTION('center_axis',(0.218508012224416,0.707106781186527,-0.672498511963977));
#36912=DIRECTION('ref_axis',(-0.951056516295154,0.,-0.309016994374947));
#36913=DIRECTION('',(-0.951056516295154,0.,-0.309016994374947));
#36914=DIRECTION('center_axis',(0.,1.,0.));
#36915=DIRECTION('ref_axis',(-0.309016994374959,0.,0.95105651629515));
#36916=DIRECTION('center_axis',(0.,-1.,0.));
#36917=DIRECTION('ref_axis',(-0.309016994374959,0.,0.95105651629515));
#36918=DIRECTION('',(0.,1.,0.));
#36919=DIRECTION('center_axis',(0.218508012224416,-0.707106781186527,-0.672498511963977));
#36920=DIRECTION('ref_axis',(-0.951056516295154,0.,-0.309016994374947));
#36921=DIRECTION('',(0.951056516295154,0.,0.309016994374947));
#36922=DIRECTION('',(-0.21850801222441,-0.707106781186566,0.672498511963938));
#36923=DIRECTION('center_axis',(0.,1.,0.));
#36924=DIRECTION('ref_axis',(-0.309016994374959,0.,0.95105651629515));
#36925=DIRECTION('center_axis',(0.309016994374947,0.,-0.951056516295154));
#36926=DIRECTION('ref_axis',(-0.951056516295154,0.,-0.309016994374947));
#70687=CARTESIAN_POINT('',(0.,0.,0.));
#70688=CARTESIAN_POINT('Origin',(-24.3512401121419,-7.2,116.813364586238));
#70689=CARTESIAN_POINT('',(-24.7247837315525,-7.2,117.848601353551));
#70690=CARTESIAN_POINT('Origin',(-24.3848650377401,-7.2,116.802439185627));
#70691=CARTESIAN_POINT('',(-24.7102863810161,-7.2,118.0328076576));
#70692=CARTESIAN_POINT('',(-24.7175350562843,-7.2,117.940704505576));
#70693=CARTESIAN_POINT('',(-23.9249439920713,-7.2,115.615772316099));
#70694=CARTESIAN_POINT('Origin',(-24.3176151865437,-7.2,116.824289986849));
#70695=CARTESIAN_POINT('Origin',(-24.3176151865437,-7.2,116.824289986849));
#70696=CARTESIAN_POINT('Origin',(-24.2897593861105,-7.2,116.833340885064));
#70697=CARTESIAN_POINT('',(-23.8511305947749,-7.2,115.578162511662));
#70698=CARTESIAN_POINT('',(-23.8880372934231,-7.2,115.596967413881));
#70699=CARTESIAN_POINT('',(-24.6726765765799,-7.2,118.106621054896));
#70700=CARTESIAN_POINT('Origin',(-24.2619035856774,-7.2,116.842391783279));
#70701=CARTESIAN_POINT('Origin',(-24.2619035856774,-7.2,116.842391783279));
#70702=CARTESIAN_POINT('Origin',(-24.3848650377401,-7.2,116.802439185627));
#70703=CARTESIAN_POINT('Origin',(-24.1807258342645,-7.2,116.868768033609));
#70704=CARTESIAN_POINT('',(-24.5321718749764,-7.2,118.226623406752));
#70705=CARTESIAN_POINT('',(-24.6024242257782,-7.2,118.166622230824));
#70706=CARTESIAN_POINT('',(-23.6669242907266,-7.2,115.563665161126));
#70707=CARTESIAN_POINT('Origin',(-24.0995480828515,-7.2,116.895144283939));
#70708=CARTESIAN_POINT('Origin',(-24.0995480828515,-7.2,116.895144283939));
#70709=CARTESIAN_POINT('Origin',(-22.8631746116678,-7.2,117.296866376627));
#70710=CARTESIAN_POINT('',(-23.381607335838,-7.2,115.656370259438));
#70711=CARTESIAN_POINT('',(-22.4305508195429,-7.2,115.965387253813));
#70712=CARTESIAN_POINT('Origin',(-23.814231127963,-7.2,116.987849382252));
#70713=CARTESIAN_POINT('Origin',(7.,-6.45,127.));
#70714=CARTESIAN_POINT('',(6.38,-6.4,127.));
#70715=CARTESIAN_POINT('Origin',(7.,-6.4,127.));
#70716=CARTESIAN_POINT('',(6.48,-6.5,127.));
#70717=CARTESIAN_POINT('',(6.43,-6.45,127.));
#70718=CARTESIAN_POINT('Origin',(7.,-6.5,127.));
#70719=CARTESIAN_POINT('Origin',(7.,-8.1,127.));
#70720=CARTESIAN_POINT('',(6.48,-7.9,127.));
#70721=CARTESIAN_POINT('Origin',(7.,-7.9,127.));
#70722=CARTESIAN_POINT('',(6.48,-8.1,127.));
#70723=CARTESIAN_POINT('Origin',(5.51247677078473,-6.4,126.411332101473));
#70724=CARTESIAN_POINT('',(4.48674914492698,-6.4,125.02678684895));
#70725=CARTESIAN_POINT('',(3.8069117573021,-6.4,127.1191111848));
#70726=CARTESIAN_POINT('',(3.93054736833321,-6.4,126.738599900121));
#70727=CARTESIAN_POINT('',(6.66008130618755,-6.4,128.046162167925));
#70728=CARTESIAN_POINT('',(3.99872699598973,-6.4,127.181435733887));
#70729=CARTESIAN_POINT('',(7.33991869381246,-6.4,125.953837832075));
#70730=CARTESIAN_POINT('Origin',(7.00000000000001,-6.4,127.));
#70731=CARTESIAN_POINT('',(6.58067741620492,-6.4,125.707145386788));
#70732=CARTESIAN_POINT('Origin',(7.,-7.95,127.));
#70733=CARTESIAN_POINT('',(6.38,-8.,127.));
#70734=CARTESIAN_POINT('Origin',(7.,-8.,127.));
#70735=CARTESIAN_POINT('',(6.43,-7.95,127.));
#70736=CARTESIAN_POINT('Origin',(5.51247677078473,-8.,126.411332101473));
#70737=CARTESIAN_POINT('',(3.8069117573021,-8.,127.1191111848));
#70738=CARTESIAN_POINT('',(4.48674914492698,-8.,125.02678684895));
#70739=CARTESIAN_POINT('',(3.93054736833321,-8.,126.738599900121));
#70740=CARTESIAN_POINT('',(7.33991869381247,-8.,125.953837832075));
#70741=CARTESIAN_POINT('',(6.58067741620492,-8.,125.707145386788));
#70742=CARTESIAN_POINT('',(6.66008130618756,-8.,128.046162167925));
#70743=CARTESIAN_POINT('Origin',(7.00000000000001,-8.,127.));
#70744=CARTESIAN_POINT('',(3.99872699598973,-8.,127.181435733887));
#70745=CARTESIAN_POINT('Origin',(-21.5792483146694,-7.2,117.714039319033));
#70746=CARTESIAN_POINT('',(-22.059424932609,-7.2,119.030067592127));
#70747=CARTESIAN_POINT('',(-21.1941773483592,-7.2,116.367109346501));
#70748=CARTESIAN_POINT('Origin',(-21.6268011404841,-7.2,117.698588469314));
#70749=CARTESIAN_POINT('Origin',(-21.6268011404841,-7.2,117.698588469314));
#70750=CARTESIAN_POINT('',(-21.933417581542,-7.2,118.965863639935));
#70751=CARTESIAN_POINT('',(-21.9964212570755,-7.2,118.997965616031));
#70752=CARTESIAN_POINT('Origin',(-21.5316954888546,-7.2,117.729490168752));
#70753=CARTESIAN_POINT('Origin',(-22.8631746116678,-7.2,117.296866376627));
#70754=CARTESIAN_POINT('',(-21.6697056065068,-7.2,116.212600849313));
#70755=CARTESIAN_POINT('Origin',(-22.1023293986317,-7.2,117.544079972127));
#70756=CARTESIAN_POINT('',(-22.4305508195429,-7.2,115.965387253813));
#70757=CARTESIAN_POINT('Origin',(-21.9643192809795,-7.2,119.060969291565));
#70758=CARTESIAN_POINT('',(-21.2226784944797,-7.2,116.778433652456));
#70759=CARTESIAN_POINT('Origin',(-21.5316954888546,-7.2,117.729490168752));
#70760=CARTESIAN_POINT('Origin',(-24.2159532206504,-7.2,118.224222853435));
#70761=CARTESIAN_POINT('',(-23.4125090352755,-7.2,115.751475911068));
#70762=CARTESIAN_POINT('Origin',(-23.814231127963,-7.2,116.987849382252));
#70763=CARTESIAN_POINT('Origin',(-23.7191254763334,-7.2,117.018751081689));
#70764=CARTESIAN_POINT('',(-23.2222977320165,-7.2,115.813279309943));
#70765=CARTESIAN_POINT('Origin',(-23.6240198247039,-7.2,117.049652781127));
#70766=CARTESIAN_POINT('',(-23.317403383646,-7.2,115.782377610505));
#70767=CARTESIAN_POINT('Origin',(-24.0720944665476,-7.2,118.428684729755));
#70768=CARTESIAN_POINT('',(-23.191396032579,-7.2,115.718173658313));
#70769=CARTESIAN_POINT('Origin',(-23.6240198247039,-7.2,117.049652781127));
#70770=CARTESIAN_POINT('Origin',(-22.8631746116678,-7.2,117.296866376627));
#70771=CARTESIAN_POINT('',(-22.6207621228019,-7.2,115.903583854938));
#70772=CARTESIAN_POINT('',(-22.4305508195429,-7.2,115.965387253813));
#70773=CARTESIAN_POINT('Origin',(-23.0533859149268,-7.2,117.235062977752));
#70774=CARTESIAN_POINT('Origin',(-23.4551080076143,-7.2,118.471436448935));
#70775=CARTESIAN_POINT('',(-22.6516638222394,-7.2,115.998689506568));
#70776=CARTESIAN_POINT('Origin',(-23.0533859149268,-7.2,117.235062977752));
#70777=CARTESIAN_POINT('Origin',(-22.9582802632973,-7.2,117.265964677189));
#70778=CARTESIAN_POINT('',(-22.4614525189804,-7.2,116.060492905443));
#70779=CARTESIAN_POINT('Origin',(-22.8631746116678,-7.2,117.296866376627));
#70780=CARTESIAN_POINT('',(-22.5565581706099,-7.2,116.029591206005));
#70781=CARTESIAN_POINT('Origin',(-23.3112492535115,-7.2,118.675898325255));
#70782=CARTESIAN_POINT('',(-22.4305508195429,-7.2,115.965387253813));
#70783=CARTESIAN_POINT('Origin',(-22.8631746116678,-7.2,117.296866376627));
#70784=CARTESIAN_POINT('Origin',(-22.8631746116678,-7.2,117.296866376627));
#70785=CARTESIAN_POINT('',(-21.8599169097658,-7.2,116.150797450438));
#70786=CARTESIAN_POINT('',(-22.4305508195429,-7.2,115.965387253813));
#70787=CARTESIAN_POINT('Origin',(-22.2925407018907,-7.2,117.482276573252));
#70788=CARTESIAN_POINT('Origin',(-22.6942627945782,-7.2,118.718650044435));
#70789=CARTESIAN_POINT('',(-21.8908186092033,-7.2,116.245903102068));
#70790=CARTESIAN_POINT('Origin',(-22.2925407018907,-7.2,117.482276573252));
#70791=CARTESIAN_POINT('Origin',(-22.1974350502612,-7.2,117.513178272689));
#70792=CARTESIAN_POINT('',(-21.7006073059442,-7.2,116.307706500943));
#70793=CARTESIAN_POINT('Origin',(-22.1023293986317,-7.2,117.544079972127));
#70794=CARTESIAN_POINT('',(-21.7957129575738,-7.2,116.276804801505));
#70795=CARTESIAN_POINT('Origin',(-22.5504040404754,-7.2,118.923111920755));
#70796=CARTESIAN_POINT('Origin',(3.68330495955212,-7.2,127.499533791318));
#70797=CARTESIAN_POINT('',(4.61035594267696,-7.2,124.646364242432));
#70798=CARTESIAN_POINT('Origin',(4.14683045111454,-7.2,126.072949016875));
#70799=CARTESIAN_POINT('',(4.51765084436447,-7.9,124.931681197321));
#70800=CARTESIAN_POINT('',(4.35541692231764,-8.42499999999998,125.430985868376));
#70801=CARTESIAN_POINT('',(3.7760100578646,-7.9,127.214216836429));
#70802=CARTESIAN_POINT('',(3.70648123413024,-7.67499999999999,127.428204552596));
#70803=CARTESIAN_POINT('',(3.7760100578646,-6.5,127.214216836429));
#70804=CARTESIAN_POINT('',(3.77601005786461,-7.6,127.214216836429));
#70805=CARTESIAN_POINT('',(3.70648123413024,-6.72500000000001,127.428204552596));
#70806=CARTESIAN_POINT('',(4.51765084436447,-6.5,124.931681197321));
#70807=CARTESIAN_POINT('',(4.35541692231764,-5.97500000000002,125.430985868376));
#70808=CARTESIAN_POINT('',(4.51765084436447,-7.6,124.931681197321));
#70809=CARTESIAN_POINT('Origin',(4.09927762529978,-7.2,126.057498167156));
#70810=CARTESIAN_POINT('',(4.54615199048493,-7.2,124.520356891365));
#70811=CARTESIAN_POINT('Origin',(4.05172479948503,-7.2,126.042047317438));
#70812=CARTESIAN_POINT('',(4.57825396658095,-7.2,124.583360566899));
#70813=CARTESIAN_POINT('Origin',(0.342604385933935,-7.2,124.836881039375));
#70814=CARTESIAN_POINT('',(-2.87208883661725,-7.2,122.110024335241));
#70815=CARTESIAN_POINT('Origin',(-3.36651602761717,-7.2,123.631714761313));
#70816=CARTESIAN_POINT('',(0.837031576933849,-7.2,123.315190613303));
#70817=CARTESIAN_POINT('Origin',(-3.41406885343193,-7.2,123.616263911594));
#70818=CARTESIAN_POINT('',(-2.99809618768428,-7.2,122.174228287433));
#70819=CARTESIAN_POINT('Origin',(-3.46162167924668,-7.2,123.600813061876));
#70820=CARTESIAN_POINT('',(-2.93509251215077,-7.2,122.142126311337));
#70821=CARTESIAN_POINT('Origin',(-3.77063867362164,-7.2,124.551869578171));
#70822=CARTESIAN_POINT('',(-3.15260468487175,-7.2,122.64975654558));
#70823=CARTESIAN_POINT('Origin',(-3.46162167924669,-7.2,123.600813061876));
#70824=CARTESIAN_POINT('Origin',(-12.4966585840506,-7.2,120.665151615314));
#70825=CARTESIAN_POINT('',(-12.1876415896757,-7.2,119.714095099018));
#70826=CARTESIAN_POINT('Origin',(3.98327614627098,-6.45,127.228988559702));
#70827=CARTESIAN_POINT('',(6.62917960675006,-6.5,128.141267819554));
#70828=CARTESIAN_POINT('',(3.96782529655224,-6.5,127.276541385517));
#70829=CARTESIAN_POINT('',(6.62917960675006,-6.5,128.141267819554));
#70830=CARTESIAN_POINT('Origin',(2.82495354156945,-8.,126.905199842054));
#70831=CARTESIAN_POINT('',(6.62917960675006,-7.9,128.141267819554));
#70832=CARTESIAN_POINT('',(3.96782529655224,-7.9,127.276541385517));
#70833=CARTESIAN_POINT('',(6.62917960675006,-8.,128.141267819554));
#70834=CARTESIAN_POINT('Origin',(3.98327614627098,-7.95,127.228988559702));
#70835=CARTESIAN_POINT('',(6.62917960675006,-7.9,128.141267819554));
#70836=CARTESIAN_POINT('Origin',(7.00000000000001,-6.45,127.));
#70837=CARTESIAN_POINT('',(7.37082039324996,-6.5,125.858732180446));
#70838=CARTESIAN_POINT('',(7.37082039324996,-6.5,125.858732180446));
#70839=CARTESIAN_POINT('Origin',(7.00000000000001,-6.5,127.));
#70840=CARTESIAN_POINT('Origin',(6.59612826592367,-6.45,125.659592560973));
#70841=CARTESIAN_POINT('',(6.61157911564241,-6.5,125.612039735158));
#70842=CARTESIAN_POINT('Origin',(7.00000000000001,-8.,127.));
#70843=CARTESIAN_POINT('',(7.37082039324996,-7.9,125.858732180446));
#70844=CARTESIAN_POINT('Origin',(7.00000000000001,-7.9,127.));
#70845=CARTESIAN_POINT('',(7.37082039324996,-8.,125.858732180446));
#70846=CARTESIAN_POINT('Origin',(6.59612826592367,-7.95,125.659592560973));
#70847=CARTESIAN_POINT('',(6.61157911564241,-7.9,125.612039735158));
#70848=CARTESIAN_POINT('',(7.37082039324996,-7.9,125.858732180446));
#70849=CARTESIAN_POINT('Origin',(7.00000000000001,-7.95,127.));
#70850=CARTESIAN_POINT('Origin',(7.37082039324994,-8.,125.858732180446));
#71469=UNCERTAINTY_MEASURE_WITH_UNIT(LENGTH_MEASURE(0.001),#71493,
'DISTANCE_ACCURACY_VALUE',
'Maximum model space distance between geometric entities at asserted c
onnectivities');
#71471=UNCERTAINTY_MEASURE_WITH_UNIT(LENGTH_MEASURE(0.001),#71493,
'DISTANCE_ACCURACY_VALUE',
'Maximum model space distance between geometric entities at asserted c
onnectivities');
#71490=(
GEOMETRIC_REPRESENTATION_CONTEXT(3)
GLOBAL_UNCERTAINTY_ASSIGNED_CONTEXT((#71469))
GLOBAL_UNIT_ASSIGNED_CONTEXT((#71493,#71495,#71496))
REPRESENTATION_CONTEXT('','3D')
);
#71492=(
GEOMETRIC_REPRESENTATION_CONTEXT(3)
GLOBAL_UNCERTAINTY_ASSIGNED_CONTEXT((#71471))
GLOBAL_UNIT_ASSIGNED_CONTEXT((#71493,#71495,#71496))
REPRESENTATION_CONTEXT('','3D')
);
#71493=(
LENGTH_UNIT()
NAMED_UNIT(*)
SI_UNIT(.CENTI.,.METRE.)
);
#71495=(
NAMED_UNIT(*)
PLANE_ANGLE_UNIT()
SI_UNIT($,.RADIAN.)
);
#71496=(
NAMED_UNIT(*)
SI_UNIT($,.STERADIAN.)
SOLID_ANGLE_UNIT()
);
#71515=SHAPE_DEFINITION_REPRESENTATION(#71535,#71620);
#71535=PRODUCT_DEFINITION_SHAPE('',$,#71641);
#71620=SHAPE_REPRESENTATION('',(#30477),#71490);
#71622=PRODUCT_DEFINITION_CONTEXT('part definition',#71684,'design');
#71641=PRODUCT_DEFINITION('2026-10-19-03-30-44-438',
'11_Pump_Operating_Handle_Arm',#71661,#71622);
#71661=PRODUCT_DEFINITION_FORMATION('',$,#71704);
#71684=APPLICATION_CONTEXT(
'Core Data for Automotive Mechanical Design Process');
#71685=PRODUCT_CONTEXT('part definition',#71684,'mechanical');
#71704=PRODUCT('2026-10-19-03-30-44-438','11_Pump_Operating_Handle_Arm',
$,(#71685));
#71874=COLOUR_RGB('Sky Blue',0.24,0.69,0.87);
#71875=FILL_AREA_STYLE_COLOUR('',#71874);
#71876=FILL_AREA_STYLE('',(#71875));
#71877=SURFACE_STYLE_FILL_AREA(#71876);
#71878=SURFACE_SIDE_STYLE('',(#71877));
#71879=SURFACE_STYLE_USAGE(.BOTH.,#71878);
#71880=PRESENTATION_STYLE_ASSIGNMENT((#71879));
ENDSEC;
END-ISO-10303-21;
